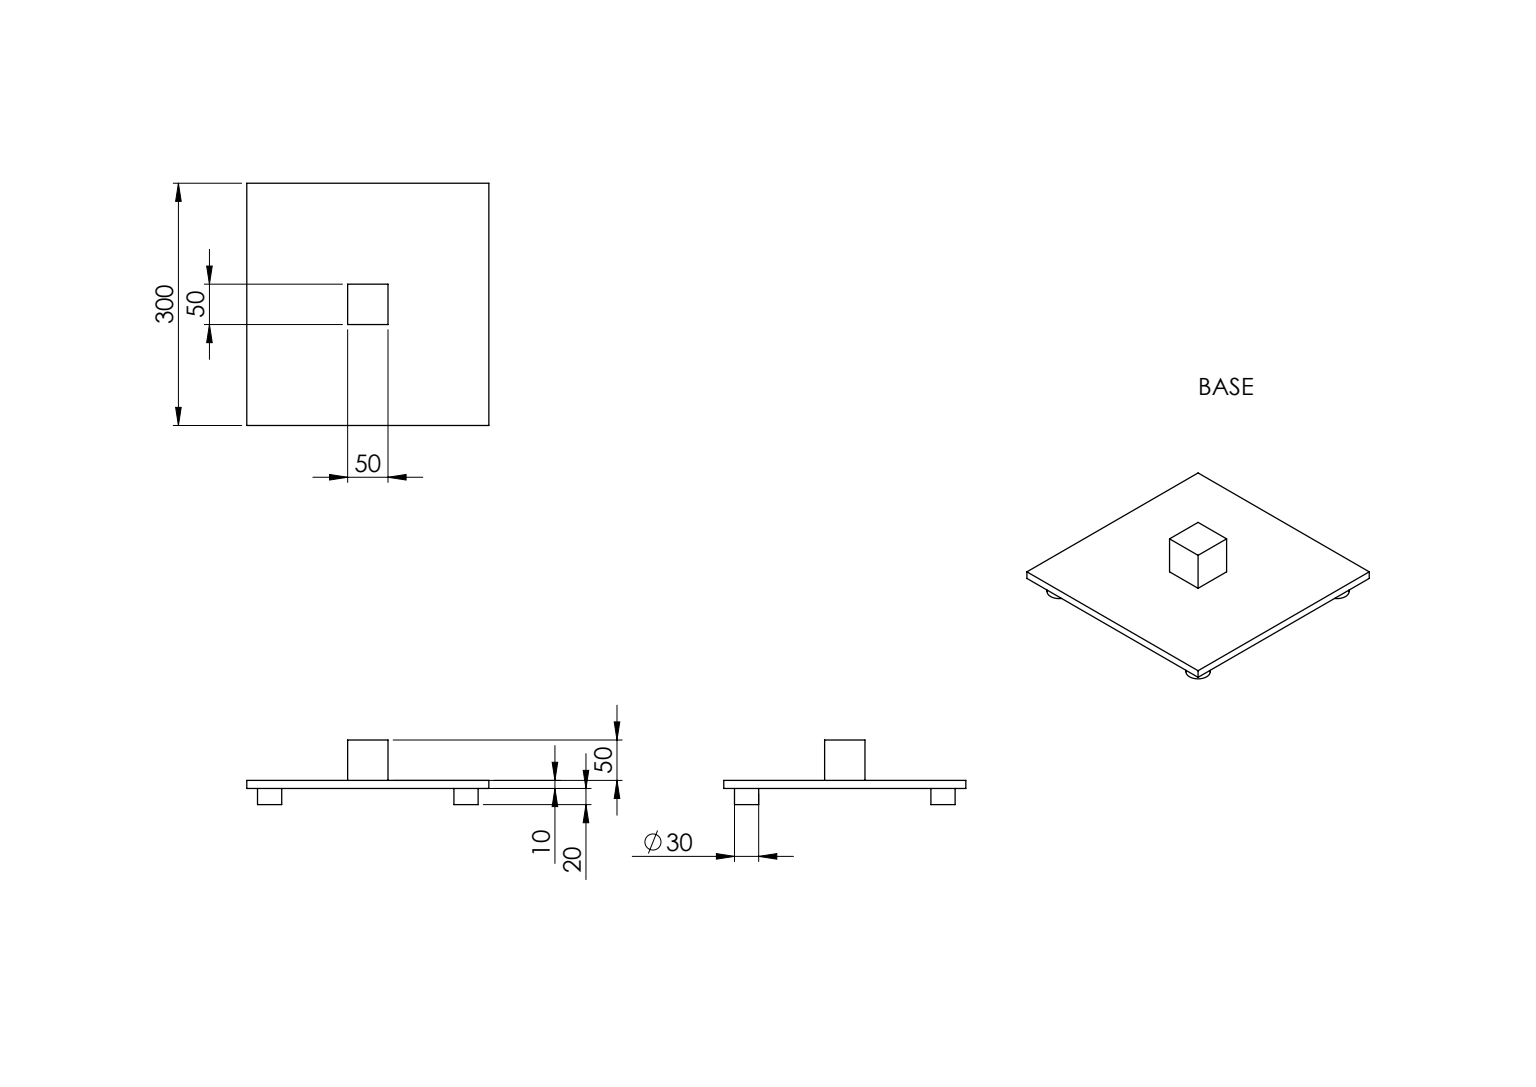
ISO-10303-21;
HEADER;
FILE_DESCRIPTION (('STEP AP214'),
    '1' );
FILE_NAME ('base.step',
    '2026-10-22T16:49:52',
    ( '' ),
    ( '' ),
    'SwSTEP 2.0',
    'SolidWorks 2026',
    '' );
FILE_SCHEMA (( 'AUTOMOTIVE_DESIGN' ));
ENDSEC;

DATA;
#2=EDGE_LOOP ( 'NONE', ( #5035, #4306, #1396, #717 ) ) ;
#9=DIRECTION ( 'NONE',  ( 1.000000000000000000, -0.000000000000000000, 0.000000000000000000 ) ) ;
#24=EDGE_LOOP ( 'NONE', ( #1798, #2180 ) ) ;
#25=CARTESIAN_POINT ( 'NONE',  ( 121.7157287525372311, 0.000000000000000000, -121.7157287525388369 ) ) ;
#29=DIRECTION ( 'NONE',  ( 0.000000000000000000, -1.000000000000000000, 0.000000000000000000 ) ) ;
#39=EDGE_CURVE ( 'NONE', #183, #4714, #3882, .T. ) ;
#40=AXIS2_PLACEMENT_3D ( 'NONE', #2568, #2148, #4717 ) ;
#42=CARTESIAN_POINT ( 'NONE',  ( 149.9999999999999716, 10.00000000000000000, 149.9999999999999716 ) ) ;
#45=EDGE_LOOP ( 'NONE', ( #4536, #2353, #4861, #2749 ) ) ;
#48=ORIENTED_EDGE ( 'NONE', *, *, #2007, .T. ) ;
#62=DIRECTION ( 'NONE',  ( -0.000000000000000000, -0.000000000000000000, 1.000000000000000000 ) ) ;
#102=CARTESIAN_POINT ( 'NONE',  ( 24.99999999999999645, 60.00000000000000711, -25.00000000000000000 ) ) ;
#108=LINE ( 'NONE', #1461, #5040 ) ;
#111=CARTESIAN_POINT ( 'NONE',  ( -150.0000000000000284, 10.00000000000000000, 149.9999999999999147 ) ) ;
#115=EDGE_CURVE ( 'NONE', #4871, #4344, #3809, .T. ) ;
#117=CARTESIAN_POINT ( 'NONE',  ( -121.7157287525381122, -20.00000000000000000, 106.7157287525380127 ) ) ;
#126=EDGE_CURVE ( 'NONE', #4344, #870, #2364, .T. ) ;
#130=AXIS2_PLACEMENT_3D ( 'NONE', #2726, #4867, #1140 ) ;
#136=EDGE_CURVE ( 'NONE', #4283, #3488, #3860, .T. ) ;
#147=CARTESIAN_POINT ( 'NONE',  ( -121.7157287525381122, 0.000000000000000000, 106.7157287525380127 ) ) ;
#154=VECTOR ( 'NONE', #5264, 1000.000000000000000 ) ;
#156=EDGE_CURVE ( 'NONE', #870, #4344, #3054, .T. ) ;
#158=LINE ( 'NONE', #4749, #4217 ) ;
#163=FACE_OUTER_BOUND ( 'NONE', #2172, .T. ) ;
#183=VERTEX_POINT ( 'NONE', #3483 ) ;
#184=CARTESIAN_POINT ( 'NONE',  ( -121.7157287525381122, 0.000000000000000000, 121.7157287525380127 ) ) ;
#188=EDGE_LOOP ( 'NONE', ( #4329, #3309, #4220, #3176 ) ) ;
#196=DIRECTION ( 'NONE',  ( -0.000000000000000000, 1.000000000000000000, -0.000000000000000000 ) ) ;
#201=CARTESIAN_POINT ( 'NONE',  ( 121.7157287525384533, -20.00000000000000000, 121.7157287525376859 ) ) ;
#212=ADVANCED_FACE ( 'NONE', ( #4821, #5247 ), #1493, .F. ) ;
#225=DIRECTION ( 'NONE',  ( -0.000000000000000000, 1.000000000000000000, -0.000000000000000000 ) ) ;
#232=VECTOR ( 'NONE', #2038, 1000.000000000000000 ) ;
#234=VECTOR ( 'NONE', #2330, 1000.000000000000000 ) ;
#254=CARTESIAN_POINT ( 'NONE',  ( -150.0000000000000284, 0.000000000000000000, 149.9999999999999147 ) ) ;
#282=LINE ( 'NONE', #1853, #2054 ) ;
#284=EDGE_CURVE ( 'NONE', #3602, #4122, #385, .T. ) ;
#285=VERTEX_POINT ( 'NONE', #3734 ) ;
#289=DIRECTION ( 'NONE',  ( 0.000000000000000000, 0.000000000000000000, 1.000000000000000000 ) ) ;
#297=DIRECTION ( 'NONE',  ( 0.000000000000000000, -1.000000000000000000, 0.000000000000000000 ) ) ;
#301=UNCERTAINTY_MEASURE_WITH_UNIT (LENGTH_MEASURE( 1.000000000000000082E-05 ), #2011, 'distance_accuracy_value', 'NONE');
#303=ORIENTED_EDGE ( 'NONE', *, *, #2481, .F. ) ;
#313=PRODUCT ( 'base', 'base', '', ( #3317 ) ) ;
#316=CARTESIAN_POINT ( 'NONE',  ( 121.7157287525384533, -20.00000000000000000, 121.7157287525376859 ) ) ;
#327=VECTOR ( 'NONE', #3004, 1000.000000000000000 ) ;
#344=FACE_OUTER_BOUND ( 'NONE', #1476, .T. ) ;
#360=ORIENTED_EDGE ( 'NONE', *, *, #1632, .T. ) ;
#377=DIRECTION ( 'NONE',  ( 0.000000000000000000, -0.000000000000000000, -1.000000000000000000 ) ) ;
#380=EDGE_CURVE ( 'NONE', #4951, #2954, #3997, .T. ) ;
#381=AXIS2_PLACEMENT_3D ( 'NONE', #2439, #1631, #3694 ) ;
#385=LINE ( 'NONE', #2047, #5346 ) ;
#392=ORIENTED_EDGE ( 'NONE', *, *, #593, .F. ) ;
#395=CIRCLE ( 'NONE', #5175, 14.99999999999998579 ) ;
#406=ORIENTED_EDGE ( 'NONE', *, *, #1500, .F. ) ;
#410=CYLINDRICAL_SURFACE ( 'NONE', #2644, 15.00000000000000000 ) ;
#420=AXIS2_PLACEMENT_3D ( 'NONE', #4558, #2003, #4859 ) ;
#430=ORIENTED_EDGE ( 'NONE', *, *, #862, .F. ) ;
#434=CARTESIAN_POINT ( 'NONE',  ( -25.00000000000000000, 60.00000000000000711, 25.00000000000000000 ) ) ;
#442=DIRECTION ( 'NONE',  ( 1.000000000000000000, 0.000000000000000000, 1.850371707708594316E-16 ) ) ;
#453=EDGE_CURVE ( 'NONE', #5233, #1447, #4280, .T. ) ;
#459=DIRECTION ( 'NONE',  ( 0.000000000000000000, -1.000000000000000000, 0.000000000000000000 ) ) ;
#462=PLANE ( 'NONE',  #2932 ) ;
#468=CIRCLE ( 'NONE', #3263, 15.00000000000000000 ) ;
#471=ADVANCED_FACE ( 'NONE', ( #519 ), #2233, .F. ) ;
#488=AXIS2_PLACEMENT_3D ( 'NONE', #3147, #2245, #5188 ) ;
#508=VERTEX_POINT ( 'NONE', #3877 ) ;
#519=FACE_OUTER_BOUND ( 'NONE', #1880, .T. ) ;
#520=CARTESIAN_POINT ( 'NONE',  ( 121.7157287525372311, -20.00000000000000000, -106.7157287525388369 ) ) ;
#523=LINE ( 'NONE', #3324, #777 ) ;
#526=CARTESIAN_POINT ( 'NONE',  ( 121.7157287525384533, -20.00000000000000000, 106.7157287525376859 ) ) ;
#529=VERTEX_POINT ( 'NONE', #4604 ) ;
#537=CARTESIAN_POINT ( 'NONE',  ( -25.00000000000000000, 10.00000000000000000, 25.00000000000000000 ) ) ;
#544=FACE_BOUND ( 'NONE', #1003, .T. ) ;
#551=CYLINDRICAL_SURFACE ( 'NONE', #3899, 15.00000000000000000 ) ;
#557=VECTOR ( 'NONE', #1931, 1000.000000000000000 ) ;
#565=PRODUCT_DEFINITION_FORMATION_WITH_SPECIFIED_SOURCE ( 'ANY', '', #313, .NOT_KNOWN. ) ;
#577=EDGE_LOOP ( 'NONE', ( #3215, #4979 ) ) ;
#589=ORIENTED_EDGE ( 'NONE', *, *, #453, .T. ) ;
#592=LINE ( 'NONE', #537, #4258 ) ;
#593=EDGE_CURVE ( 'NONE', #285, #2404, #4298, .T. ) ;
#595=ORIENTED_EDGE ( 'NONE', *, *, #3799, .F. ) ;
#596=DIRECTION ( 'NONE',  ( 0.000000000000000000, -1.000000000000000000, 0.000000000000000000 ) ) ;
#598=CARTESIAN_POINT ( 'NONE',  ( 121.7157287525384533, -20.00000000000000000, 106.7157287525376859 ) ) ;
#603=CARTESIAN_POINT ( 'NONE',  ( 25.00000000000000355, 60.00000000000000711, 25.00000000000000000 ) ) ;
#611=EDGE_CURVE ( 'NONE', #4353, #4532, #731, .T. ) ;
#623=DIRECTION ( 'NONE',  ( -1.000000000000000000, -0.000000000000000000, -0.000000000000000000 ) ) ;
#634=FACE_OUTER_BOUND ( 'NONE', #1339, .T. ) ;
#649=DIRECTION ( 'NONE',  ( 1.000000000000000000, 0.000000000000000000, -0.000000000000000000 ) ) ;
#656=VERTEX_POINT ( 'NONE', #3193 ) ;
#664=( GEOMETRIC_REPRESENTATION_CONTEXT ( 3 ) GLOBAL_UNCERTAINTY_ASSIGNED_CONTEXT ( ( #4876 ) ) GLOBAL_UNIT_ASSIGNED_CONTEXT ( ( #2048, #3372, #4579 ) ) REPRESENTATION_CONTEXT ( 'NONE', 'WORKASPACE' ) );
#665=EDGE_CURVE ( 'NONE', #5319, #2146, #4998, .T. ) ;
#685=CARTESIAN_POINT ( 'NONE',  ( 0.000000000000000000, 0.000000000000000000, 0.000000000000000000 ) ) ;
#694=DIRECTION ( 'NONE',  ( -1.000000000000000000, 0.000000000000000000, -0.000000000000000000 ) ) ;
#701=VERTEX_POINT ( 'NONE', #3518 ) ;
#703=CARTESIAN_POINT ( 'NONE',  ( -121.7157287525392917, 0.000000000000000000, -121.7157287525368332 ) ) ;
#707=( NAMED_UNIT ( * ) PLANE_ANGLE_UNIT ( ) SI_UNIT ( $, .RADIAN. ) );
#717=ORIENTED_EDGE ( 'NONE', *, *, #4118, .T. ) ;
#719=FACE_OUTER_BOUND ( 'NONE', #24, .T. ) ;
#731=CIRCLE ( 'NONE', #1938, 15.00000000000000000 ) ;
#736=CARTESIAN_POINT ( 'NONE',  ( 121.7157287525384533, 0.000000000000000000, 136.7157287525376717 ) ) ;
#738=CYLINDRICAL_SURFACE ( 'NONE', #1107, 15.00000000000000000 ) ;
#747=DIRECTION ( 'NONE',  ( 0.000000000000000000, 0.000000000000000000, 1.000000000000000000 ) ) ;
#756=CARTESIAN_POINT ( 'NONE',  ( -121.7157287525392917, -20.00000000000000000, -121.7157287525368332 ) ) ;
#769=DIRECTION ( 'NONE',  ( 1.000000000000000000, 0.000000000000000000, 0.000000000000000000 ) ) ;
#775=DIRECTION ( 'NONE',  ( 0.000000000000000000, -1.000000000000000000, 0.000000000000000000 ) ) ;
#777=VECTOR ( 'NONE', #442, 1000.000000000000000 ) ;
#799=DIRECTION ( 'NONE',  ( -1.000000000000000000, 0.000000000000000000, -9.251858538542972814E-17 ) ) ;
#804=DIRECTION ( 'NONE',  ( 0.000000000000000000, -0.000000000000000000, -1.000000000000000000 ) ) ;
#813=VERTEX_POINT ( 'NONE', #2815 ) ;
#826=AXIS2_PLACEMENT_3D ( 'NONE', #3603, #1034, #1920 ) ;
#842=EDGE_CURVE ( 'NONE', #3267, #4388, #3750, .T. ) ;
#847=AXIS2_PLACEMENT_3D ( 'NONE', #2606, #3446, #2183 ) ;
#848=ADVANCED_FACE ( 'NONE', ( #4987 ), #410, .T. ) ;
#854=DIRECTION ( 'NONE',  ( 0.000000000000000000, 0.000000000000000000, -1.000000000000000000 ) ) ;
#862=EDGE_CURVE ( 'NONE', #4388, #5233, #1567, .T. ) ;
#870=VERTEX_POINT ( 'NONE', #736 ) ;
#889=CARTESIAN_POINT ( 'NONE',  ( 0.000000000000000000, 60.00000000000000711, 0.000000000000000000 ) ) ;
#903=ORIENTED_EDGE ( 'NONE', *, *, #2485, .F. ) ;
#904=DIRECTION ( 'NONE',  ( 0.000000000000000000, 0.000000000000000000, -1.000000000000000000 ) ) ;
#908=EDGE_CURVE ( 'NONE', #4532, #4353, #4554, .T. ) ;
#917=PLANE ( 'NONE',  #130 ) ;
#925=ORIENTED_EDGE ( 'NONE', *, *, #5286, .F. ) ;
#936=VECTOR ( 'NONE', #623, 1000.000000000000000 ) ;
#938=EDGE_CURVE ( 'NONE', #3516, #2213, #468, .T. ) ;
#947=DIRECTION ( 'NONE',  ( -1.000000000000000000, 0.000000000000000000, 0.000000000000000000 ) ) ;
#955=DIRECTION ( 'NONE',  ( 0.000000000000000000, -1.000000000000000000, 0.000000000000000000 ) ) ;
#959=DIRECTION ( 'NONE',  ( -0.000000000000000000, -0.000000000000000000, 1.000000000000000000 ) ) ;
#962=VECTOR ( 'NONE', #3089, 1000.000000000000000 ) ;
#972=DIRECTION ( 'NONE',  ( -1.000000000000000000, -0.000000000000000000, -2.775557561562891351E-16 ) ) ;
#974=ORIENTED_EDGE ( 'NONE', *, *, #39, .F. ) ;
#979=PRODUCT_DEFINITION ( 'UNKNOWN', '', #565, #1182 ) ;
#997=AXIS2_PLACEMENT_3D ( 'NONE', #201, #1860, #5201 ) ;
#1003=EDGE_LOOP ( 'NONE', ( #4168, #2495 ) ) ;
#1006=CARTESIAN_POINT ( 'NONE',  ( 121.7157287525372311, -20.00000000000000000, -121.7157287525388369 ) ) ;
#1008=PLANE ( 'NONE',  #1116 ) ;
#1016=DIRECTION ( 'NONE',  ( 0.000000000000000000, 0.000000000000000000, -1.000000000000000000 ) ) ;
#1025=CARTESIAN_POINT ( 'NONE',  ( -121.7157287525381122, -20.00000000000000000, 121.7157287525380127 ) ) ;
#1029=EDGE_CURVE ( 'NONE', #2213, #3516, #1411, .T. ) ;
#1032=DIRECTION ( 'NONE',  ( -0.000000000000000000, 1.000000000000000000, -0.000000000000000000 ) ) ;
#1033=ORIENTED_EDGE ( 'NONE', *, *, #1852, .T. ) ;
#1034=DIRECTION ( 'NONE',  ( 0.000000000000000000, -1.000000000000000000, 0.000000000000000000 ) ) ;
#1035=CARTESIAN_POINT ( 'NONE',  ( -121.7157287525392917, -20.00000000000000000, -106.7157287525368332 ) ) ;
#1042=LINE ( 'NONE', #2710, #936 ) ;
#1045=EDGE_LOOP ( 'NONE', ( #5269, #1939, #430, #4843 ) ) ;
#1067=CARTESIAN_POINT ( 'NONE',  ( -121.7157287525381122, -20.00000000000000000, 106.7157287525380127 ) ) ;
#1081=EDGE_CURVE ( 'NONE', #4871, #529, #4303, .T. ) ;
#1085=ADVANCED_FACE ( 'NONE', ( #5203 ), #3984, .T. ) ;
#1088=DIRECTION ( 'NONE',  ( 0.000000000000000000, 0.000000000000000000, 1.000000000000000000 ) ) ;
#1089=FACE_OUTER_BOUND ( 'NONE', #4892, .T. ) ;
#1095=ORIENTED_EDGE ( 'NONE', *, *, #380, .F. ) ;
#1106=EDGE_CURVE ( 'NONE', #3488, #2372, #158, .T. ) ;
#1107=AXIS2_PLACEMENT_3D ( 'NONE', #3670, #2761, #1088 ) ;
#1116=AXIS2_PLACEMENT_3D ( 'NONE', #2685, #1433, #649 ) ;
#1117=ORIENTED_EDGE ( 'NONE', *, *, #39, .T. ) ;
#1132=CYLINDRICAL_SURFACE ( 'NONE', #4647, 15.00000000000000000 ) ;
#1140=DIRECTION ( 'NONE',  ( 0.000000000000000000, -0.000000000000000000, -1.000000000000000000 ) ) ;
#1166=AXIS2_PLACEMENT_3D ( 'NONE', #1842, #297, #2681 ) ;
#1168=( NAMED_UNIT ( * ) SI_UNIT ( $, .STERADIAN. ) SOLID_ANGLE_UNIT ( ) );
#1171=ORIENTED_EDGE ( 'NONE', *, *, #4109, .F. ) ;
#1182=PRODUCT_DEFINITION_CONTEXT ( 'detailed design', #4958, 'design' ) ;
#1206=LINE ( 'NONE', #2980, #232 ) ;
#1213=DIRECTION ( 'NONE',  ( 0.000000000000000000, -1.000000000000000000, 0.000000000000000000 ) ) ;
#1237=ORIENTED_EDGE ( 'NONE', *, *, #1632, .F. ) ;
#1250=DIRECTION ( 'NONE',  ( 0.000000000000000000, 0.000000000000000000, 1.000000000000000000 ) ) ;
#1273=ORIENTED_EDGE ( 'NONE', *, *, #1106, .T. ) ;
#1288=VECTOR ( 'NONE', #2476, 1000.000000000000000 ) ;
#1293=ORIENTED_EDGE ( 'NONE', *, *, #4109, .T. ) ;
#1299=CARTESIAN_POINT ( 'NONE',  ( 121.7157287525372311, -20.00000000000000000, -121.7157287525388369 ) ) ;
#1307=EDGE_LOOP ( 'NONE', ( #4818, #5283 ) ) ;
#1313=ADVANCED_FACE ( 'NONE', ( #5047 ), #462, .T. ) ;
#1319=ORIENTED_EDGE ( 'NONE', *, *, #908, .F. ) ;
#1320=CYLINDRICAL_SURFACE ( 'NONE', #3962, 15.00000000000000000 ) ;
#1334=VECTOR ( 'NONE', #3501, 1000.000000000000000 ) ;
#1338=CARTESIAN_POINT ( 'NONE',  ( 121.7157287525384533, 0.000000000000000000, 106.7157287525376859 ) ) ;
#1339=EDGE_LOOP ( 'NONE', ( #2416, #2759, #4548, #5314 ) ) ;
#1354=PRODUCT_DEFINITION_SHAPE ( 'NONE', 'NONE',  #979 ) ;
#1356=DIRECTION ( 'NONE',  ( 0.000000000000000000, -0.000000000000000000, -1.000000000000000000 ) ) ;
#1361=VECTOR ( 'NONE', #3225, 1000.000000000000000 ) ;
#1372=EDGE_LOOP ( 'NONE', ( #4478, #589, #4101, #1914 ) ) ;
#1377=EDGE_LOOP ( 'NONE', ( #2702, #5065, #3631, #3686 ) ) ;
#1380=DIRECTION ( 'NONE',  ( -2.775557561562891351E-16, 0.000000000000000000, 1.000000000000000000 ) ) ;
#1391=EDGE_LOOP ( 'NONE', ( #4455, #5173, #2058, #4539 ) ) ;
#1396=ORIENTED_EDGE ( 'NONE', *, *, #453, .F. ) ;
#1399=EDGE_CURVE ( 'NONE', #656, #2372, #5132, .T. ) ;
#1411=CIRCLE ( 'NONE', #5004, 15.00000000000000000 ) ;
#1413=LINE ( 'NONE', #2595, #4663 ) ;
#1419=CARTESIAN_POINT ( 'NONE',  ( 121.7157287525372311, -20.00000000000000000, -121.7157287525388369 ) ) ;
#1422=DIRECTION ( 'NONE',  ( -0.000000000000000000, -0.000000000000000000, 1.000000000000000000 ) ) ;
#1425=AXIS2_PLACEMENT_3D ( 'NONE', #1666, #2967, #4606 ) ;
#1432=DIRECTION ( 'NONE',  ( 0.000000000000000000, 0.000000000000000000, -1.000000000000000000 ) ) ;
#1433=DIRECTION ( 'NONE',  ( 0.000000000000000000, 0.000000000000000000, 1.000000000000000000 ) ) ;
#1445=LINE ( 'NONE', #1912, #3386 ) ;
#1447=VERTEX_POINT ( 'NONE', #4703 ) ;
#1450=ORIENTED_EDGE ( 'NONE', *, *, #4120, .F. ) ;
#1460=DIRECTION ( 'NONE',  ( 0.000000000000000000, 0.000000000000000000, -1.000000000000000000 ) ) ;
#1461=CARTESIAN_POINT ( 'NONE',  ( 149.9999999999999716, 0.000000000000000000, 149.9999999999999716 ) ) ;
#1463=LINE ( 'NONE', #3039, #2746 ) ;
#1476=EDGE_LOOP ( 'NONE', ( #3157, #4991, #5195, #4804 ) ) ;
#1479=DIRECTION ( 'NONE',  ( 1.000000000000000000, 0.000000000000000000, 1.850371707708594316E-16 ) ) ;
#1493=PLANE ( 'NONE',  #3592 ) ;
#1496=EDGE_CURVE ( 'NONE', #2213, #4532, #2628, .T. ) ;
#1499=CYLINDRICAL_SURFACE ( 'NONE', #4583, 15.00000000000000000 ) ;
#1500=EDGE_CURVE ( 'NONE', #2146, #4714, #1463, .T. ) ;
#1501=ORIENTED_EDGE ( 'NONE', *, *, #3927, .T. ) ;
#1514=FACE_BOUND ( 'NONE', #4193, .T. ) ;
#1529=MECHANICAL_DESIGN_GEOMETRIC_PRESENTATION_REPRESENTATION('',(#3380),#664);
#1530=CARTESIAN_POINT ( 'NONE',  ( -25.00000000000000000, 10.00000000000000000, 25.00000000000000000 ) ) ;
#1537=DIRECTION ( 'NONE',  ( 0.000000000000000000, -1.000000000000000000, 0.000000000000000000 ) ) ;
#1541=FILL_AREA_STYLE ('',( #4043 ) ) ;
#1559=CARTESIAN_POINT ( 'NONE',  ( -150.0000000000000284, 10.00000000000000000, 149.9999999999999147 ) ) ;
#1567=LINE ( 'NONE', #4930, #3867 ) ;
#1573=ADVANCED_FACE ( 'NONE', ( #719 ), #2415, .T. ) ;
#1582=DIRECTION ( 'NONE',  ( 0.000000000000000000, -1.000000000000000000, 0.000000000000000000 ) ) ;
#1590=( NAMED_UNIT ( * ) PLANE_ANGLE_UNIT ( ) SI_UNIT ( $, .RADIAN. ) );
#1598=CARTESIAN_POINT ( 'NONE',  ( 121.7157287525372311, 0.000000000000000000, -121.7157287525388369 ) ) ;
#1605=CARTESIAN_POINT ( 'NONE',  ( 25.00000000000000355, 10.00000000000000000, 25.00000000000000000 ) ) ;
#1609=CIRCLE ( 'NONE', #4230, 14.99999999999998579 ) ;
#1618=AXIS2_PLACEMENT_3D ( 'NONE', #4282, #2205, #1460 ) ;
#1623=ORIENTED_EDGE ( 'NONE', *, *, #3900, .F. ) ;
#1631=DIRECTION ( 'NONE',  ( 0.000000000000000000, -1.000000000000000000, 0.000000000000000000 ) ) ;
#1632=EDGE_CURVE ( 'NONE', #2355, #3602, #3201, .T. ) ;
#1646=CARTESIAN_POINT ( 'NONE',  ( 121.7157287525372311, 0.000000000000000000, -106.7157287525388369 ) ) ;
#1666=CARTESIAN_POINT ( 'NONE',  ( 0.000000000000000000, 10.00000000000000000, 0.000000000000000000 ) ) ;
#1698=CIRCLE ( 'NONE', #1948, 14.99999999999998579 ) ;
#1700=COLOUR_RGB ( '',0.8941176470588234615, 0.8941176470588234615, 0.8941176470588234615 ) ;
#1704=CLOSED_SHELL ( 'NONE', ( #4182, #4266, #848, #2419, #4143, #3046, #3376, #3139, #5154, #3778, #3323, #3865, #1313, #4477, #5357, #1813, #1573, #2678, #1085, #3540, #4827, #2531, #212, #1733, #471 ) ) ;
#1731=CARTESIAN_POINT ( 'NONE',  ( 25.00000000000000355, 60.00000000000000711, 25.00000000000000000 ) ) ;
#1733=ADVANCED_FACE ( 'NONE', ( #3490 ), #2567, .F. ) ;
#1739=CARTESIAN_POINT ( 'NONE',  ( -121.7157287525381122, -20.00000000000000000, 121.7157287525380127 ) ) ;
#1768=DIRECTION ( 'NONE',  ( 9.251858538542972814E-17, 0.000000000000000000, -1.000000000000000000 ) ) ;
#1769=AXIS2_PLACEMENT_3D ( 'NONE', #3034, #4675, #947 ) ;
#1772=DIRECTION ( 'NONE',  ( 0.000000000000000000, -1.000000000000000000, 0.000000000000000000 ) ) ;
#1774=PLANE ( 'NONE',  #4397 ) ;
#1777=VECTOR ( 'NONE', #5215, 1000.000000000000000 ) ;
#1782=( GEOMETRIC_REPRESENTATION_CONTEXT ( 3 ) GLOBAL_UNCERTAINTY_ASSIGNED_CONTEXT ( ( #301 ) ) GLOBAL_UNIT_ASSIGNED_CONTEXT ( ( #2011, #1590, #4806 ) ) REPRESENTATION_CONTEXT ( 'NONE', 'WORKASPACE' ) );
#1796=LINE ( 'NONE', #520, #3389 ) ;
#1798=ORIENTED_EDGE ( 'NONE', *, *, #2100, .T. ) ;
#1806=CARTESIAN_POINT ( 'NONE',  ( 121.7157287525384533, -20.00000000000000000, 136.7157287525376717 ) ) ;
#1813=ADVANCED_FACE ( 'NONE', ( #4863 ), #1320, .T. ) ;
#1827=EDGE_CURVE ( 'NONE', #701, #3600, #3182, .T. ) ;
#1831=LINE ( 'NONE', #3148, #234 ) ;
#1840=DIRECTION ( 'NONE',  ( -0.000000000000000000, -0.000000000000000000, 1.000000000000000000 ) ) ;
#1841=EDGE_LOOP ( 'NONE', ( #1033, #2082 ) ) ;
#1842=CARTESIAN_POINT ( 'NONE',  ( -121.7157287525392917, -20.00000000000000000, -121.7157287525368332 ) ) ;
#1848=DIRECTION ( 'NONE',  ( -1.000000000000000000, 0.000000000000000000, 1.387778780781445676E-16 ) ) ;
#1852=EDGE_CURVE ( 'NONE', #529, #4871, #2843, .T. ) ;
#1853=CARTESIAN_POINT ( 'NONE',  ( 25.00000000000000355, 60.00000000000000711, 25.00000000000000000 ) ) ;
#1860=DIRECTION ( 'NONE',  ( 0.000000000000000000, -1.000000000000000000, 0.000000000000000000 ) ) ;
#1877=ORIENTED_EDGE ( 'NONE', *, *, #842, .F. ) ;
#1880=EDGE_LOOP ( 'NONE', ( #925, #1095, #4640, #392 ) ) ;
#1887=CARTESIAN_POINT ( 'NONE',  ( -25.00000000000000000, 60.00000000000000711, 25.00000000000000000 ) ) ;
#1891=ORIENTED_EDGE ( 'NONE', *, *, #284, .F. ) ;
#1901=LINE ( 'NONE', #2406, #2958 ) ;
#1909=CYLINDRICAL_SURFACE ( 'NONE', #488, 15.00000000000000000 ) ;
#1912=CARTESIAN_POINT ( 'NONE',  ( 24.99999999999999645, 60.00000000000000711, -25.00000000000000000 ) ) ;
#1914=ORIENTED_EDGE ( 'NONE', *, *, #842, .T. ) ;
#1916=AXIS2_PLACEMENT_3D ( 'NONE', #3041, #955, #4289 ) ;
#1920=DIRECTION ( 'NONE',  ( 0.000000000000000000, -0.000000000000000000, -1.000000000000000000 ) ) ;
#1927=CARTESIAN_POINT ( 'NONE',  ( -25.00000000000000000, 60.00000000000000711, 25.00000000000000000 ) ) ;
#1931=DIRECTION ( 'NONE',  ( 1.000000000000000000, 0.000000000000000000, 0.000000000000000000 ) ) ;
#1937=EDGE_LOOP ( 'NONE', ( #4559, #1171, #5244, #1501 ) ) ;
#1938=AXIS2_PLACEMENT_3D ( 'NONE', #184, #596, #2260 ) ;
#1939=ORIENTED_EDGE ( 'NONE', *, *, #4118, .F. ) ;
#1947=EDGE_LOOP ( 'NONE', ( #2453, #4214, #4944, #595 ) ) ;
#1948=AXIS2_PLACEMENT_3D ( 'NONE', #25, #4893, #2807 ) ;
#1986=CARTESIAN_POINT ( 'NONE',  ( 121.7157287525372311, -20.00000000000000000, -121.7157287525388369 ) ) ;
#1987=DIRECTION ( 'NONE',  ( -0.000000000000000000, -1.000000000000000000, -0.000000000000000000 ) ) ;
#2003=DIRECTION ( 'NONE',  ( -0.000000000000000000, 1.000000000000000000, -0.000000000000000000 ) ) ;
#2004=ORIENTED_EDGE ( 'NONE', *, *, #3841, .F. ) ;
#2007=EDGE_CURVE ( 'NONE', #5319, #183, #3244, .T. ) ;
#2010=ORIENTED_EDGE ( 'NONE', *, *, #611, .F. ) ;
#2011=( LENGTH_UNIT ( ) NAMED_UNIT ( * ) SI_UNIT ( .MILLI., .METRE. ) );
#2030=EDGE_CURVE ( 'NONE', #2382, #813, #1698, .T. ) ;
#2037=DIRECTION ( 'NONE',  ( -0.000000000000000000, 1.000000000000000000, -0.000000000000000000 ) ) ;
#2038=DIRECTION ( 'NONE',  ( -0.000000000000000000, -1.000000000000000000, -0.000000000000000000 ) ) ;
#2039=DIRECTION ( 'NONE',  ( -9.251858538542972814E-17, 0.000000000000000000, 1.000000000000000000 ) ) ;
#2042=UNCERTAINTY_MEASURE_WITH_UNIT (LENGTH_MEASURE( 1.000000000000000082E-05 ), #4102, 'distance_accuracy_value', 'NONE');
#2044=VECTOR ( 'NONE', #4121, 1000.000000000000000 ) ;
#2046=ORIENTED_EDGE ( 'NONE', *, *, #3190, .T. ) ;
#2047=CARTESIAN_POINT ( 'NONE',  ( 25.00000000000000355, 10.00000000000000000, 25.00000000000000000 ) ) ;
#2048=( LENGTH_UNIT ( ) NAMED_UNIT ( * ) SI_UNIT ( .MILLI., .METRE. ) );
#2054=VECTOR ( 'NONE', #2249, 1000.000000000000000 ) ;
#2058=ORIENTED_EDGE ( 'NONE', *, *, #3438, .T. ) ;
#2082=ORIENTED_EDGE ( 'NONE', *, *, #1081, .T. ) ;
#2099=LINE ( 'NONE', #4994, #3097 ) ;
#2100=EDGE_CURVE ( 'NONE', #4209, #3573, #395, .T. ) ;
#2123=DIRECTION ( 'NONE',  ( -1.000000000000000000, -0.000000000000000000, -0.000000000000000000 ) ) ;
#2146=VERTEX_POINT ( 'NONE', #2537 ) ;
#2148=DIRECTION ( 'NONE',  ( 0.000000000000000000, -1.000000000000000000, 0.000000000000000000 ) ) ;
#2162=VECTOR ( 'NONE', #2123, 1000.000000000000000 ) ;
#2172=EDGE_LOOP ( 'NONE', ( #1273, #3625, #2342, #2767 ) ) ;
#2180=ORIENTED_EDGE ( 'NONE', *, *, #3245, .T. ) ;
#2183=DIRECTION ( 'NONE',  ( -1.000000000000000000, 0.000000000000000000, 0.000000000000000000 ) ) ;
#2205=DIRECTION ( 'NONE',  ( 0.000000000000000000, -1.000000000000000000, 0.000000000000000000 ) ) ;
#2213=VERTEX_POINT ( 'NONE', #117 ) ;
#2233=CYLINDRICAL_SURFACE ( 'NONE', #3417, 6.499999999999983125 ) ;
#2245=DIRECTION ( 'NONE',  ( -0.000000000000000000, 1.000000000000000000, -0.000000000000000000 ) ) ;
#2249=DIRECTION ( 'NONE',  ( -0.000000000000000000, -1.000000000000000000, -0.000000000000000000 ) ) ;
#2250=DIRECTION ( 'NONE',  ( 1.000000000000000000, 0.000000000000000000, 0.000000000000000000 ) ) ;
#2260=DIRECTION ( 'NONE',  ( 0.000000000000000000, 0.000000000000000000, -1.000000000000000000 ) ) ;
#2267=CARTESIAN_POINT ( 'NONE',  ( 149.9999999999999716, 10.00000000000000000, 149.9999999999999716 ) ) ;
#2282=LINE ( 'NONE', #4671, #3311 ) ;
#2283=EDGE_CURVE ( 'NONE', #4388, #3602, #282, .T. ) ;
#2286=ORIENTED_EDGE ( 'NONE', *, *, #1399, .T. ) ;
#2330=DIRECTION ( 'NONE',  ( -0.000000000000000000, -0.000000000000000000, 1.000000000000000000 ) ) ;
#2332=DIRECTION ( 'NONE',  ( 0.000000000000000000, 0.000000000000000000, 1.000000000000000000 ) ) ;
#2342=ORIENTED_EDGE ( 'NONE', *, *, #4716, .F. ) ;
#2350=LINE ( 'NONE', #1927, #154 ) ;
#2353=ORIENTED_EDGE ( 'NONE', *, *, #136, .F. ) ;
#2354=CARTESIAN_POINT ( 'NONE',  ( -25.00000000000000000, 10.00000000000000000, 25.00000000000000000 ) ) ;
#2355=VERTEX_POINT ( 'NONE', #1530 ) ;
#2361=FACE_OUTER_BOUND ( 'NONE', #3559, .T. ) ;
#2362=EDGE_LOOP ( 'NONE', ( #974, #2920 ) ) ;
#2364=CIRCLE ( 'NONE', #2804, 15.00000000000000000 ) ;
#2372=VERTEX_POINT ( 'NONE', #3326 ) ;
#2382=VERTEX_POINT ( 'NONE', #1646 ) ;
#2389=DIRECTION ( 'NONE',  ( 0.000000000000000000, 0.000000000000000000, 1.000000000000000000 ) ) ;
#2404=VERTEX_POINT ( 'NONE', #2425 ) ;
#2406=CARTESIAN_POINT ( 'NONE',  ( 150.0000000000000000, 10.00000000000000000, -150.0000000000000000 ) ) ;
#2415=PLANE ( 'NONE',  #5008 ) ;
#2416=ORIENTED_EDGE ( 'NONE', *, *, #4972, .F. ) ;
#2419=ADVANCED_FACE ( 'NONE', ( #344 ), #1132, .T. ) ;
#2421=CIRCLE ( 'NONE', #847, 6.499999999999983125 ) ;
#2425=CARTESIAN_POINT ( 'NONE',  ( 6.499999999999981348, 35.00000000000000000, 25.00000000000000000 ) ) ;
#2426=CYLINDRICAL_SURFACE ( 'NONE', #420, 15.00000000000000000 ) ;
#2427=EDGE_LOOP ( 'NONE', ( #3156, #4006 ) ) ;
#2429=VECTOR ( 'NONE', #959, 1000.000000000000000 ) ;
#2434=CARTESIAN_POINT ( 'NONE',  ( 0.000000000000000000, 0.000000000000000000, 0.000000000000000000 ) ) ;
#2439=CARTESIAN_POINT ( 'NONE',  ( -121.7157287525381122, 0.000000000000000000, 121.7157287525380127 ) ) ;
#2442=DIRECTION ( 'NONE',  ( 0.000000000000000000, 0.000000000000000000, 1.000000000000000000 ) ) ;
#2453=ORIENTED_EDGE ( 'NONE', *, *, #3245, .F. ) ;
#2458=APPLICATION_CONTEXT ( 'automotive_design' ) ;
#2469=DIRECTION ( 'NONE',  ( 1.000000000000000000, 0.000000000000000000, 0.000000000000000000 ) ) ;
#2476=DIRECTION ( 'NONE',  ( -0.000000000000000000, -0.000000000000000000, 1.000000000000000000 ) ) ;
#2478=VERTEX_POINT ( 'NONE', #5337 ) ;
#2481=EDGE_CURVE ( 'NONE', #2146, #5319, #1609, .T. ) ;
#2484=SHAPE_REPRESENTATION_RELATIONSHIP ( 'NONE' , 'NONE' ,  #3706, #2946 ) ;
#2485=EDGE_CURVE ( 'NONE', #656, #701, #4587, .T. ) ;
#2488=DIRECTION ( 'NONE',  ( 1.000000000000000000, 0.000000000000000000, 0.000000000000000000 ) ) ;
#2491=FACE_OUTER_BOUND ( 'NONE', #45, .T. ) ;
#2495=ORIENTED_EDGE ( 'NONE', *, *, #4972, .T. ) ;
#2498=CARTESIAN_POINT ( 'NONE',  ( -6.499999999999984901, 35.00000000000000000, -25.00000000000000000 ) ) ;
#2514=EDGE_LOOP ( 'NONE', ( #360, #2646, #1877, #1293 ) ) ;
#2519=ORIENTED_EDGE ( 'NONE', *, *, #4887, .T. ) ;
#2530=DIRECTION ( 'NONE',  ( 0.000000000000000000, 0.000000000000000000, -1.000000000000000000 ) ) ;
#2531=ADVANCED_FACE ( 'NONE', ( #2585 ), #1774, .F. ) ;
#2537=CARTESIAN_POINT ( 'NONE',  ( -121.7157287525392917, -20.00000000000000000, -136.7157287525368474 ) ) ;
#2565=ORIENTED_EDGE ( 'NONE', *, *, #3260, .F. ) ;
#2567=PLANE ( 'NONE',  #4064 ) ;
#2568=CARTESIAN_POINT ( 'NONE',  ( 121.7157287525384533, -20.00000000000000000, 121.7157287525376859 ) ) ;
#2585=FACE_OUTER_BOUND ( 'NONE', #1937, .T. ) ;
#2595=CARTESIAN_POINT ( 'NONE',  ( -150.0000000000000284, 10.00000000000000000, -150.0000000000000853 ) ) ;
#2603=CARTESIAN_POINT ( 'NONE',  ( -1.676835913137321903E-15, 35.00000000000000000, 30.00000000000000711 ) ) ;
#2606=CARTESIAN_POINT ( 'NONE',  ( -1.676835913137321903E-15, 35.00000000000000000, 25.00000000000000000 ) ) ;
#2628=LINE ( 'NONE', #1067, #1777 ) ;
#2633=FACE_OUTER_BOUND ( 'NONE', #1391, .T. ) ;
#2644=AXIS2_PLACEMENT_3D ( 'NONE', #1986, #2037, #1250 ) ;
#2646=ORIENTED_EDGE ( 'NONE', *, *, #2283, .F. ) ;
#2657=CARTESIAN_POINT ( 'NONE',  ( -150.0000000000000284, 0.000000000000000000, 149.9999999999999147 ) ) ;
#2678=ADVANCED_FACE ( 'NONE', ( #5219 ), #1909, .T. ) ;
#2681=DIRECTION ( 'NONE',  ( 0.000000000000000000, 0.000000000000000000, -1.000000000000000000 ) ) ;
#2682=DIRECTION ( 'NONE',  ( 1.850371707708594316E-16, 0.000000000000000000, -1.000000000000000000 ) ) ;
#2685=CARTESIAN_POINT ( 'NONE',  ( -25.00000000000000000, 60.00000000000000711, -25.00000000000000000 ) ) ;
#2691=FACE_OUTER_BOUND ( 'NONE', #1045, .T. ) ;
#2698=DIRECTION ( 'NONE',  ( -0.000000000000000000, -0.000000000000000000, 1.000000000000000000 ) ) ;
#2701=DIRECTION ( 'NONE',  ( -1.000000000000000000, -0.000000000000000000, -2.775557561562891351E-16 ) ) ;
#2702=ORIENTED_EDGE ( 'NONE', *, *, #1496, .F. ) ;
#2710=CARTESIAN_POINT ( 'NONE',  ( -25.00000000000000000, 10.00000000000000000, -25.00000000000000000 ) ) ;
#2726=CARTESIAN_POINT ( 'NONE',  ( 121.7157287525384533, -20.00000000000000000, 121.7157287525376859 ) ) ;
#2746=VECTOR ( 'NONE', #3144, 1000.000000000000000 ) ;
#2749=ORIENTED_EDGE ( 'NONE', *, *, #4120, .T. ) ;
#2759=ORIENTED_EDGE ( 'NONE', *, *, #5286, .T. ) ;
#2761=DIRECTION ( 'NONE',  ( -0.000000000000000000, 1.000000000000000000, -0.000000000000000000 ) ) ;
#2767=ORIENTED_EDGE ( 'NONE', *, *, #136, .T. ) ;
#2797=CARTESIAN_POINT ( 'NONE',  ( -150.0000000000000284, 10.00000000000000000, -150.0000000000000853 ) ) ;
#2804=AXIS2_PLACEMENT_3D ( 'NONE', #4734, #1772, #1016 ) ;
#2807=DIRECTION ( 'NONE',  ( 0.000000000000000000, 0.000000000000000000, -1.000000000000000000 ) ) ;
#2815=CARTESIAN_POINT ( 'NONE',  ( 121.7157287525372311, 0.000000000000000000, -136.7157287525388085 ) ) ;
#2843=CIRCLE ( 'NONE', #997, 15.00000000000000000 ) ;
#2849=MECHANICAL_DESIGN_GEOMETRIC_PRESENTATION_REPRESENTATION('',(#4730),#1782);
#2850=DIRECTION ( 'NONE',  ( 0.000000000000000000, 0.000000000000000000, -1.000000000000000000 ) ) ;
#2870=AXIS2_PLACEMENT_3D ( 'NONE', #3824, #2698, #2250 ) ;
#2884=FACE_BOUND ( 'NONE', #4150, .T. ) ;
#2914=DIRECTION ( 'NONE',  ( 0.000000000000000000, -1.000000000000000000, 0.000000000000000000 ) ) ;
#2920=ORIENTED_EDGE ( 'NONE', *, *, #3190, .F. ) ;
#2925=EDGE_LOOP ( 'NONE', ( #4124, #1450, #4407, #3749 ) ) ;
#2932=AXIS2_PLACEMENT_3D ( 'NONE', #3419, #4183, #1356 ) ;
#2941=AXIS2_PLACEMENT_3D ( 'NONE', #703, #1537, #2530 ) ;
#2946=ADVANCED_BREP_SHAPE_REPRESENTATION ( '', ( #3645, #4154 ), #3368 ) ;
#2954=VERTEX_POINT ( 'NONE', #2498 ) ;
#2958=VECTOR ( 'NONE', #1987, 1000.000000000000000 ) ;
#2960=ORIENTED_EDGE ( 'NONE', *, *, #2007, .F. ) ;
#2967=DIRECTION ( 'NONE',  ( 0.000000000000000000, -1.000000000000000000, 0.000000000000000000 ) ) ;
#2968=EDGE_CURVE ( 'NONE', #3516, #4353, #2099, .T. ) ;
#2971=DIRECTION ( 'NONE',  ( 1.000000000000000000, -0.000000000000000000, 0.000000000000000000 ) ) ;
#2975=DIRECTION ( 'NONE',  ( 0.000000000000000000, 0.000000000000000000, -1.000000000000000000 ) ) ;
#2980=CARTESIAN_POINT ( 'NONE',  ( -25.00000000000000000, 60.00000000000000711, -25.00000000000000000 ) ) ;
#2983=EDGE_CURVE ( 'NONE', #2404, #285, #2421, .T. ) ;
#2997=CARTESIAN_POINT ( 'NONE',  ( -121.7157287525381122, 0.000000000000000000, 136.7157287525380127 ) ) ;
#3004=DIRECTION ( 'NONE',  ( -0.000000000000000000, -1.000000000000000000, -0.000000000000000000 ) ) ;
#3016=DIRECTION ( 'NONE',  ( 0.000000000000000000, 0.000000000000000000, -1.000000000000000000 ) ) ;
#3026=AXIS2_PLACEMENT_3D ( 'NONE', #3904, #2682, #3496 ) ;
#3033=ORIENTED_EDGE ( 'NONE', *, *, #1827, .T. ) ;
#3034=CARTESIAN_POINT ( 'NONE',  ( -1.676835913137321903E-15, 35.00000000000000000, 25.00000000000000000 ) ) ;
#3036=CARTESIAN_POINT ( 'NONE',  ( -150.0000000000000284, 10.00000000000000000, -150.0000000000000853 ) ) ;
#3039=CARTESIAN_POINT ( 'NONE',  ( -121.7157287525392917, -20.00000000000000000, -136.7157287525368190 ) ) ;
#3041=CARTESIAN_POINT ( 'NONE',  ( 121.7157287525384533, 0.000000000000000000, 121.7157287525376859 ) ) ;
#3046=ADVANCED_FACE ( 'NONE', ( #4551, #4264 ), #5028, .F. ) ;
#3054=CIRCLE ( 'NONE', #1916, 15.00000000000000000 ) ;
#3056=ORIENTED_EDGE ( 'NONE', *, *, #156, .F. ) ;
#3058=CARTESIAN_POINT ( 'NONE',  ( -25.00000000000000000, 60.00000000000000711, -25.00000000000000000 ) ) ;
#3059=CARTESIAN_POINT ( 'NONE',  ( -150.0000000000000284, 0.000000000000000000, -150.0000000000000853 ) ) ;
#3089=DIRECTION ( 'NONE',  ( -0.000000000000000000, 1.000000000000000000, -0.000000000000000000 ) ) ;
#3095=DIRECTION ( 'NONE',  ( -0.000000000000000000, -1.000000000000000000, -0.000000000000000000 ) ) ;
#3097=VECTOR ( 'NONE', #3804, 1000.000000000000000 ) ;
#3105=AXIS2_PLACEMENT_3D ( 'NONE', #603, #1848, #3528 ) ;
#3132=ORIENTED_EDGE ( 'NONE', *, *, #1106, .F. ) ;
#3139=ADVANCED_FACE ( 'NONE', ( #3581 ), #4787, .F. ) ;
#3144=DIRECTION ( 'NONE',  ( -0.000000000000000000, 1.000000000000000000, -0.000000000000000000 ) ) ;
#3147=CARTESIAN_POINT ( 'NONE',  ( -121.7157287525392917, -20.00000000000000000, -121.7157287525368332 ) ) ;
#3148=CARTESIAN_POINT ( 'NONE',  ( 6.499999999999981348, 35.00000000000000000, 30.00000000000000711 ) ) ;
#3156=ORIENTED_EDGE ( 'NONE', *, *, #665, .T. ) ;
#3157=ORIENTED_EDGE ( 'NONE', *, *, #1081, .F. ) ;
#3168=DIRECTION ( 'NONE',  ( 0.000000000000000000, 0.000000000000000000, -1.000000000000000000 ) ) ;
#3176=ORIENTED_EDGE ( 'NONE', *, *, #2968, .F. ) ;
#3182=LINE ( 'NONE', #4778, #5012 ) ;
#3190=EDGE_CURVE ( 'NONE', #4714, #183, #5190, .T. ) ;
#3193=CARTESIAN_POINT ( 'NONE',  ( 149.9999999999999716, 10.00000000000000000, 149.9999999999999716 ) ) ;
#3200=VECTOR ( 'NONE', #5218, 1000.000000000000000 ) ;
#3201=LINE ( 'NONE', #2354, #557 ) ;
#3215=ORIENTED_EDGE ( 'NONE', *, *, #2983, .T. ) ;
#3222=SURFACE_SIDE_STYLE ('',( #3692 ) ) ;
#3223=EDGE_LOOP ( 'NONE', ( #2004, #3413, #4678, #3541 ) ) ;
#3224=DIRECTION ( 'NONE',  ( -1.387778780781445676E-16, 0.000000000000000000, -1.000000000000000000 ) ) ;
#3225=DIRECTION ( 'NONE',  ( -0.000000000000000000, 1.000000000000000000, -0.000000000000000000 ) ) ;
#3237=CARTESIAN_POINT ( 'NONE',  ( -150.0000000000000284, 10.00000000000000000, 149.9999999999999147 ) ) ;
#3244=LINE ( 'NONE', #3332, #2044 ) ;
#3245=EDGE_CURVE ( 'NONE', #3573, #4209, #3543, .T. ) ;
#3260=EDGE_CURVE ( 'NONE', #813, #2382, #4658, .T. ) ;
#3263=AXIS2_PLACEMENT_3D ( 'NONE', #1739, #29, #3846 ) ;
#3267=VERTEX_POINT ( 'NONE', #3284 ) ;
#3284=CARTESIAN_POINT ( 'NONE',  ( -25.00000000000000000, 60.00000000000000711, 25.00000000000000000 ) ) ;
#3309=ORIENTED_EDGE ( 'NONE', *, *, #1496, .T. ) ;
#3311=VECTOR ( 'NONE', #1840, 1000.000000000000000 ) ;
#3317=PRODUCT_CONTEXT ( 'NONE', #2458, 'mechanical' ) ;
#3323=ADVANCED_FACE ( 'NONE', ( #4521, #3608, #1514, #2884, #1089 ), #4495, .T. ) ;
#3324=CARTESIAN_POINT ( 'NONE',  ( -150.0000000000000284, 10.00000000000000000, 149.9999999999999147 ) ) ;
#3326=CARTESIAN_POINT ( 'NONE',  ( 149.9999999999999716, 0.000000000000000000, 149.9999999999999716 ) ) ;
#3327=CARTESIAN_POINT ( 'NONE',  ( 121.7157287525372311, -20.00000000000000000, -106.7157287525388369 ) ) ;
#3332=CARTESIAN_POINT ( 'NONE',  ( -121.7157287525392917, -20.00000000000000000, -106.7157287525368332 ) ) ;
#3368=( GEOMETRIC_REPRESENTATION_CONTEXT ( 3 ) GLOBAL_UNCERTAINTY_ASSIGNED_CONTEXT ( ( #2042 ) ) GLOBAL_UNIT_ASSIGNED_CONTEXT ( ( #4102, #707, #1168 ) ) REPRESENTATION_CONTEXT ( 'NONE', 'WORKASPACE' ) );
#3372=( NAMED_UNIT ( * ) PLANE_ANGLE_UNIT ( ) SI_UNIT ( $, .RADIAN. ) );
#3376=ADVANCED_FACE ( 'NONE', ( #4413 ), #4023, .F. ) ;
#3377=ORIENTED_EDGE ( 'NONE', *, *, #2485, .T. ) ;
#3380=STYLED_ITEM('',(#5405),#3645);
#3386=VECTOR ( 'NONE', #3596, 1000.000000000000000 ) ;
#3389=VECTOR ( 'NONE', #4337, 1000.000000000000000 ) ;
#3397=AXIS2_PLACEMENT_3D ( 'NONE', #4992, #747, #2469 ) ;
#3413=ORIENTED_EDGE ( 'NONE', *, *, #2100, .F. ) ;
#3417=AXIS2_PLACEMENT_3D ( 'NONE', #2603, #62, #4696 ) ;
#3419=CARTESIAN_POINT ( 'NONE',  ( -121.7157287525381122, -20.00000000000000000, 121.7157287525380127 ) ) ;
#3438=EDGE_CURVE ( 'NONE', #529, #870, #3561, .T. ) ;
#3446=DIRECTION ( 'NONE',  ( 0.000000000000000000, 0.000000000000000000, -1.000000000000000000 ) ) ;
#3455=DIRECTION ( 'NONE',  ( -0.000000000000000000, -1.000000000000000000, -0.000000000000000000 ) ) ;
#3457=DIRECTION ( 'NONE',  ( 9.251858538542972814E-17, 0.000000000000000000, -1.000000000000000000 ) ) ;
#3465=VECTOR ( 'NONE', #972, 1000.000000000000000 ) ;
#3474=LINE ( 'NONE', #3059, #3465 ) ;
#3483=CARTESIAN_POINT ( 'NONE',  ( -121.7157287525392917, 0.000000000000000000, -106.7157287525368332 ) ) ;
#3488=VERTEX_POINT ( 'NONE', #2657 ) ;
#3490=FACE_OUTER_BOUND ( 'NONE', #1372, .T. ) ;
#3496=DIRECTION ( 'NONE',  ( -1.000000000000000000, 0.000000000000000000, -1.850371707708594316E-16 ) ) ;
#3501=DIRECTION ( 'NONE',  ( -0.000000000000000000, -1.000000000000000000, -0.000000000000000000 ) ) ;
#3516=VERTEX_POINT ( 'NONE', #4766 ) ;
#3518=CARTESIAN_POINT ( 'NONE',  ( 150.0000000000000000, 10.00000000000000000, -150.0000000000000000 ) ) ;
#3528=DIRECTION ( 'NONE',  ( 1.387778780781445676E-16, 0.000000000000000000, 1.000000000000000000 ) ) ;
#3540=ADVANCED_FACE ( 'NONE', ( #2691 ), #4347, .F. ) ;
#3541=ORIENTED_EDGE ( 'NONE', *, *, #2030, .T. ) ;
#3543=CIRCLE ( 'NONE', #3808, 14.99999999999998579 ) ;
#3559=EDGE_LOOP ( 'NONE', ( #303, #3977, #2046, #2960 ) ) ;
#3561=LINE ( 'NONE', #1806, #3200 ) ;
#3573=VERTEX_POINT ( 'NONE', #4030 ) ;
#3577=EDGE_LOOP ( 'NONE', ( #2519, #1623, #903, #2286 ) ) ;
#3581=FACE_OUTER_BOUND ( 'NONE', #2925, .T. ) ;
#3592=AXIS2_PLACEMENT_3D ( 'NONE', #5273, #3168, #694 ) ;
#3596=DIRECTION ( 'NONE',  ( -0.000000000000000000, -1.000000000000000000, -0.000000000000000000 ) ) ;
#3600=VERTEX_POINT ( 'NONE', #2797 ) ;
#3602=VERTEX_POINT ( 'NONE', #1605 ) ;
#3603=CARTESIAN_POINT ( 'NONE',  ( -121.7157287525392917, -20.00000000000000000, -121.7157287525368332 ) ) ;
#3608=FACE_BOUND ( 'NONE', #5155, .T. ) ;
#3625=ORIENTED_EDGE ( 'NONE', *, *, #1399, .F. ) ;
#3631=ORIENTED_EDGE ( 'NONE', *, *, #2968, .T. ) ;
#3640=VERTEX_POINT ( 'NONE', #4502 ) ;
#3645=MANIFOLD_SOLID_BREP ( 'Boss-Extrude3', #1704 ) ;
#3647=AXIS2_PLACEMENT_3D ( 'NONE', #685, #775, #377 ) ;
#3662=AXIS2_PLACEMENT_3D ( 'NONE', #3753, #9, #854 ) ;
#3670=CARTESIAN_POINT ( 'NONE',  ( -121.7157287525381122, -20.00000000000000000, 121.7157287525380127 ) ) ;
#3680=VECTOR ( 'NONE', #3455, 1000.000000000000000 ) ;
#3686=ORIENTED_EDGE ( 'NONE', *, *, #611, .T. ) ;
#3692=SURFACE_STYLE_FILL_AREA ( #1541 ) ;
#3694=DIRECTION ( 'NONE',  ( 0.000000000000000000, 0.000000000000000000, -1.000000000000000000 ) ) ;
#3706=SHAPE_REPRESENTATION ( 'base', ( #4154 ), #3368 ) ;
#3734=CARTESIAN_POINT ( 'NONE',  ( -6.499999999999984901, 35.00000000000000000, 25.00000000000000000 ) ) ;
#3749=ORIENTED_EDGE ( 'NONE', *, *, #3900, .T. ) ;
#3750=LINE ( 'NONE', #434, #3789 ) ;
#3753=CARTESIAN_POINT ( 'NONE',  ( -150.0000000000000284, 10.00000000000000000, 149.9999999999999147 ) ) ;
#3778=ADVANCED_FACE ( 'NONE', ( #163 ), #3931, .F. ) ;
#3787=EDGE_LOOP ( 'NONE', ( #3377, #3033, #5010, #4835 ) ) ;
#3789=VECTOR ( 'NONE', #2488, 1000.000000000000000 ) ;
#3790=DIRECTION ( 'NONE',  ( 0.000000000000000000, -1.000000000000000000, 0.000000000000000000 ) ) ;
#3795=DIRECTION ( 'NONE',  ( 0.000000000000000000, 0.000000000000000000, -1.000000000000000000 ) ) ;
#3799=EDGE_CURVE ( 'NONE', #4209, #2382, #1796, .T. ) ;
#3804=DIRECTION ( 'NONE',  ( -0.000000000000000000, 1.000000000000000000, -0.000000000000000000 ) ) ;
#3808=AXIS2_PLACEMENT_3D ( 'NONE', #1006, #5178, #1432 ) ;
#3809=LINE ( 'NONE', #526, #962 ) ;
#3814=EDGE_CURVE ( 'NONE', #508, #2478, #3474, .T. ) ;
#3824=CARTESIAN_POINT ( 'NONE',  ( -1.676835913137321903E-15, 35.00000000000000000, 30.00000000000000711 ) ) ;
#3841=EDGE_CURVE ( 'NONE', #3573, #813, #4494, .T. ) ;
#3846=DIRECTION ( 'NONE',  ( 0.000000000000000000, 0.000000000000000000, -1.000000000000000000 ) ) ;
#3860=LINE ( 'NONE', #111, #3680 ) ;
#3865=ADVANCED_FACE ( 'NONE', ( #4022 ), #738, .T. ) ;
#3867=VECTOR ( 'NONE', #3224, 1000.000000000000000 ) ;
#3877=CARTESIAN_POINT ( 'NONE',  ( 150.0000000000000000, 0.000000000000000000, -150.0000000000000000 ) ) ;
#3882=CIRCLE ( 'NONE', #2941, 14.99999999999998579 ) ;
#3899=AXIS2_PLACEMENT_3D ( 'NONE', #5189, #225, #3916 ) ;
#3900=EDGE_CURVE ( 'NONE', #701, #508, #1901, .T. ) ;
#3904=CARTESIAN_POINT ( 'NONE',  ( -150.0000000000000284, 10.00000000000000000, 149.9999999999999147 ) ) ;
#3916=DIRECTION ( 'NONE',  ( 0.000000000000000000, 0.000000000000000000, 1.000000000000000000 ) ) ;
#3927=EDGE_CURVE ( 'NONE', #1447, #3640, #1206, .T. ) ;
#3931=PLANE ( 'NONE',  #3026 ) ;
#3962=AXIS2_PLACEMENT_3D ( 'NONE', #1419, #1032, #289 ) ;
#3967=LINE ( 'NONE', #254, #2429 ) ;
#3977=ORIENTED_EDGE ( 'NONE', *, *, #1500, .T. ) ;
#3984=PLANE ( 'NONE',  #826 ) ;
#3997=CIRCLE ( 'NONE', #3397, 6.499999999999983125 ) ;
#4006=ORIENTED_EDGE ( 'NONE', *, *, #2481, .T. ) ;
#4022=FACE_OUTER_BOUND ( 'NONE', #1377, .T. ) ;
#4023=PLANE ( 'NONE',  #4582 ) ;
#4024=CARTESIAN_POINT ( 'NONE',  ( -1.676835913137321903E-15, 35.00000000000000000, -25.00000000000000000 ) ) ;
#4030=CARTESIAN_POINT ( 'NONE',  ( 121.7157287525372311, -20.00000000000000000, -136.7157287525388085 ) ) ;
#4043=FILL_AREA_STYLE_COLOUR ( '', #1700 ) ;
#4053=ORIENTED_EDGE ( 'NONE', *, *, #4953, .F. ) ;
#4062=DIRECTION ( 'NONE',  ( -0.000000000000000000, 1.000000000000000000, -0.000000000000000000 ) ) ;
#4064=AXIS2_PLACEMENT_3D ( 'NONE', #889, #2914, #4547 ) ;
#4071=DIRECTION ( 'NONE',  ( -1.387778780781445676E-16, 0.000000000000000000, -1.000000000000000000 ) ) ;
#4101=ORIENTED_EDGE ( 'NONE', *, *, #5050, .T. ) ;
#4102=( LENGTH_UNIT ( ) NAMED_UNIT ( * ) SI_UNIT ( .MILLI., .METRE. ) );
#4109=EDGE_CURVE ( 'NONE', #3267, #2355, #5068, .T. ) ;
#4118=EDGE_CURVE ( 'NONE', #5233, #4122, #1445, .T. ) ;
#4120=EDGE_CURVE ( 'NONE', #3600, #2478, #1413, .T. ) ;
#4121=DIRECTION ( 'NONE',  ( -0.000000000000000000, 1.000000000000000000, -0.000000000000000000 ) ) ;
#4122=VERTEX_POINT ( 'NONE', #5252 ) ;
#4124=ORIENTED_EDGE ( 'NONE', *, *, #3814, .T. ) ;
#4143=ADVANCED_FACE ( 'NONE', ( #4256 ), #1499, .T. ) ;
#4150=EDGE_LOOP ( 'NONE', ( #2010, #1319 ) ) ;
#4154=AXIS2_PLACEMENT_3D ( 'NONE', #2434, #5290, #769 ) ;
#4168=ORIENTED_EDGE ( 'NONE', *, *, #380, .T. ) ;
#4182=ADVANCED_FACE ( 'NONE', ( #634 ), #4426, .F. ) ;
#4183=DIRECTION ( 'NONE',  ( 0.000000000000000000, -1.000000000000000000, 0.000000000000000000 ) ) ;
#4193=EDGE_LOOP ( 'NONE', ( #3056, #5176 ) ) ;
#4198=CARTESIAN_POINT ( 'NONE',  ( -121.7157287525381122, -20.00000000000000000, 121.7157287525380127 ) ) ;
#4209=VERTEX_POINT ( 'NONE', #3327 ) ;
#4214=ORIENTED_EDGE ( 'NONE', *, *, #3841, .T. ) ;
#4217=VECTOR ( 'NONE', #1479, 1000.000000000000000 ) ;
#4220=ORIENTED_EDGE ( 'NONE', *, *, #908, .T. ) ;
#4226=PLANE ( 'NONE',  #3662 ) ;
#4230=AXIS2_PLACEMENT_3D ( 'NONE', #756, #1582, #904 ) ;
#4237=EDGE_CURVE ( 'NONE', #3600, #4283, #5280, .T. ) ;
#4256=FACE_OUTER_BOUND ( 'NONE', #188, .T. ) ;
#4258=VECTOR ( 'NONE', #1422, 1000.000000000000000 ) ;
#4264=FACE_BOUND ( 'NONE', #5216, .T. ) ;
#4266=ADVANCED_FACE ( 'NONE', ( #2361 ), #2426, .T. ) ;
#4280=LINE ( 'NONE', #3058, #2162 ) ;
#4282=CARTESIAN_POINT ( 'NONE',  ( -121.7157287525392917, 0.000000000000000000, -121.7157287525368332 ) ) ;
#4283=VERTEX_POINT ( 'NONE', #1559 ) ;
#4289=DIRECTION ( 'NONE',  ( 0.000000000000000000, 0.000000000000000000, -1.000000000000000000 ) ) ;
#4298=CIRCLE ( 'NONE', #1769, 6.499999999999983125 ) ;
#4303=CIRCLE ( 'NONE', #40, 15.00000000000000000 ) ;
#4306=ORIENTED_EDGE ( 'NONE', *, *, #3927, .F. ) ;
#4329=ORIENTED_EDGE ( 'NONE', *, *, #1029, .F. ) ;
#4337=DIRECTION ( 'NONE',  ( -0.000000000000000000, 1.000000000000000000, -0.000000000000000000 ) ) ;
#4344=VERTEX_POINT ( 'NONE', #1338 ) ;
#4347=PLANE ( 'NONE',  #3105 ) ;
#4353=VERTEX_POINT ( 'NONE', #2997 ) ;
#4388=VERTEX_POINT ( 'NONE', #1731 ) ;
#4397=AXIS2_PLACEMENT_3D ( 'NONE', #4685, #2971, #3016 ) ;
#4407=ORIENTED_EDGE ( 'NONE', *, *, #1827, .F. ) ;
#4413=FACE_OUTER_BOUND ( 'NONE', #3577, .T. ) ;
#4426=CYLINDRICAL_SURFACE ( 'NONE', #2870, 6.499999999999983125 ) ;
#4455=ORIENTED_EDGE ( 'NONE', *, *, #115, .F. ) ;
#4458=SURFACE_STYLE_USAGE ( .BOTH. , #3222 ) ;
#4473=EDGE_CURVE ( 'NONE', #2478, #3488, #3967, .T. ) ;
#4477=ADVANCED_FACE ( 'NONE', ( #2633 ), #551, .T. ) ;
#4478=ORIENTED_EDGE ( 'NONE', *, *, #862, .T. ) ;
#4483=VECTOR ( 'NONE', #3457, 1000.000000000000000 ) ;
#4490=AXIS2_PLACEMENT_3D ( 'NONE', #1598, #5237, #2850 ) ;
#4494=LINE ( 'NONE', #4785, #1361 ) ;
#4495=PLANE ( 'NONE',  #3647 ) ;
#4502=CARTESIAN_POINT ( 'NONE',  ( -25.00000000000000000, 10.00000000000000000, -25.00000000000000000 ) ) ;
#4516=ORIENTED_EDGE ( 'NONE', *, *, #3814, .F. ) ;
#4521=FACE_BOUND ( 'NONE', #2362, .T. ) ;
#4532=VERTEX_POINT ( 'NONE', #147 ) ;
#4536=ORIENTED_EDGE ( 'NONE', *, *, #4473, .T. ) ;
#4539=ORIENTED_EDGE ( 'NONE', *, *, #156, .T. ) ;
#4547=DIRECTION ( 'NONE',  ( 0.000000000000000000, 0.000000000000000000, -1.000000000000000000 ) ) ;
#4548=ORIENTED_EDGE ( 'NONE', *, *, #2983, .F. ) ;
#4551=FACE_OUTER_BOUND ( 'NONE', #3787, .T. ) ;
#4554=CIRCLE ( 'NONE', #381, 15.00000000000000000 ) ;
#4558=CARTESIAN_POINT ( 'NONE',  ( -121.7157287525392917, -20.00000000000000000, -121.7157287525368332 ) ) ;
#4559=ORIENTED_EDGE ( 'NONE', *, *, #5238, .T. ) ;
#4564=EDGE_CURVE ( 'NONE', #4951, #2404, #1831, .T. ) ;
#4579=( NAMED_UNIT ( * ) SI_UNIT ( $, .STERADIAN. ) SOLID_ANGLE_UNIT ( ) );
#4582=AXIS2_PLACEMENT_3D ( 'NONE', #4901, #799, #2039 ) ;
#4583=AXIS2_PLACEMENT_3D ( 'NONE', #1025, #196, #2332 ) ;
#4587=LINE ( 'NONE', #42, #4483 ) ;
#4604=CARTESIAN_POINT ( 'NONE',  ( 121.7157287525384533, -20.00000000000000000, 136.7157287525376717 ) ) ;
#4606=DIRECTION ( 'NONE',  ( 0.000000000000000000, -0.000000000000000000, -1.000000000000000000 ) ) ;
#4609=ORIENTED_EDGE ( 'NONE', *, *, #5238, .F. ) ;
#4640=ORIENTED_EDGE ( 'NONE', *, *, #4564, .T. ) ;
#4647=AXIS2_PLACEMENT_3D ( 'NONE', #316, #4062, #2389 ) ;
#4658=CIRCLE ( 'NONE', #4490, 14.99999999999998579 ) ;
#4663=VECTOR ( 'NONE', #3095, 1000.000000000000000 ) ;
#4671=CARTESIAN_POINT ( 'NONE',  ( -6.499999999999984901, 35.00000000000000000, 30.00000000000000711 ) ) ;
#4675=DIRECTION ( 'NONE',  ( 0.000000000000000000, 0.000000000000000000, -1.000000000000000000 ) ) ;
#4678=ORIENTED_EDGE ( 'NONE', *, *, #3799, .T. ) ;
#4685=CARTESIAN_POINT ( 'NONE',  ( -25.00000000000000000, 60.00000000000000711, 25.00000000000000000 ) ) ;
#4696=DIRECTION ( 'NONE',  ( 1.000000000000000000, 0.000000000000000000, 0.000000000000000000 ) ) ;
#4703=CARTESIAN_POINT ( 'NONE',  ( -25.00000000000000000, 60.00000000000000711, -25.00000000000000000 ) ) ;
#4714=VERTEX_POINT ( 'NONE', #5029 ) ;
#4716=EDGE_CURVE ( 'NONE', #4283, #656, #523, .T. ) ;
#4717=DIRECTION ( 'NONE',  ( 0.000000000000000000, 0.000000000000000000, -1.000000000000000000 ) ) ;
#4730=STYLED_ITEM ( 'NONE', ( #5320 ), #2946 ) ;
#4734=CARTESIAN_POINT ( 'NONE',  ( 121.7157287525384533, 0.000000000000000000, 121.7157287525376859 ) ) ;
#4749=CARTESIAN_POINT ( 'NONE',  ( -150.0000000000000284, 0.000000000000000000, 149.9999999999999147 ) ) ;
#4752=CIRCLE ( 'NONE', #5205, 6.499999999999983125 ) ;
#4760=CARTESIAN_POINT ( 'NONE',  ( 6.499999999999981348, 35.00000000000000000, -25.00000000000000000 ) ) ;
#4766=CARTESIAN_POINT ( 'NONE',  ( -121.7157287525381122, -20.00000000000000000, 136.7157287525380127 ) ) ;
#4778=CARTESIAN_POINT ( 'NONE',  ( -150.0000000000000284, 10.00000000000000000, -150.0000000000000853 ) ) ;
#4785=CARTESIAN_POINT ( 'NONE',  ( 121.7157287525372311, -20.00000000000000000, -136.7157287525388085 ) ) ;
#4787=PLANE ( 'NONE',  #5376 ) ;
#4804=ORIENTED_EDGE ( 'NONE', *, *, #3438, .F. ) ;
#4806=( NAMED_UNIT ( * ) SI_UNIT ( $, .STERADIAN. ) SOLID_ANGLE_UNIT ( ) );
#4818=ORIENTED_EDGE ( 'NONE', *, *, #938, .T. ) ;
#4821=FACE_BOUND ( 'NONE', #577, .T. ) ;
#4827=ADVANCED_FACE ( 'NONE', ( #544, #5129 ), #1008, .F. ) ;
#4835=ORIENTED_EDGE ( 'NONE', *, *, #4716, .T. ) ;
#4843=ORIENTED_EDGE ( 'NONE', *, *, #2283, .T. ) ;
#4859=DIRECTION ( 'NONE',  ( 0.000000000000000000, 0.000000000000000000, 1.000000000000000000 ) ) ;
#4861=ORIENTED_EDGE ( 'NONE', *, *, #4237, .F. ) ;
#4863=FACE_OUTER_BOUND ( 'NONE', #3223, .T. ) ;
#4867=DIRECTION ( 'NONE',  ( 0.000000000000000000, -1.000000000000000000, 0.000000000000000000 ) ) ;
#4871=VERTEX_POINT ( 'NONE', #598 ) ;
#4876=UNCERTAINTY_MEASURE_WITH_UNIT (LENGTH_MEASURE( 1.000000000000000082E-05 ), #2048, 'distance_accuracy_value', 'NONE');
#4887=EDGE_CURVE ( 'NONE', #2372, #508, #108, .T. ) ;
#4892=EDGE_LOOP ( 'NONE', ( #5341, #3132, #4907, #4516 ) ) ;
#4893=DIRECTION ( 'NONE',  ( 0.000000000000000000, -1.000000000000000000, 0.000000000000000000 ) ) ;
#4901=CARTESIAN_POINT ( 'NONE',  ( 149.9999999999999716, 10.00000000000000000, 149.9999999999999716 ) ) ;
#4907=ORIENTED_EDGE ( 'NONE', *, *, #4473, .F. ) ;
#4930=CARTESIAN_POINT ( 'NONE',  ( 25.00000000000000355, 60.00000000000000711, 25.00000000000000000 ) ) ;
#4936=SHAPE_DEFINITION_REPRESENTATION ( #1354, #3706 ) ;
#4944=ORIENTED_EDGE ( 'NONE', *, *, #3260, .T. ) ;
#4951=VERTEX_POINT ( 'NONE', #4760 ) ;
#4953=EDGE_CURVE ( 'NONE', #4122, #3640, #1042, .T. ) ;
#4958=APPLICATION_CONTEXT ( 'automotive_design' ) ;
#4972=EDGE_CURVE ( 'NONE', #2954, #4951, #4752, .T. ) ;
#4979=ORIENTED_EDGE ( 'NONE', *, *, #593, .T. ) ;
#4987=FACE_OUTER_BOUND ( 'NONE', #1947, .T. ) ;
#4991=ORIENTED_EDGE ( 'NONE', *, *, #115, .T. ) ;
#4992=CARTESIAN_POINT ( 'NONE',  ( -1.676835913137321903E-15, 35.00000000000000000, -25.00000000000000000 ) ) ;
#4994=CARTESIAN_POINT ( 'NONE',  ( -121.7157287525381122, -20.00000000000000000, 136.7157287525380127 ) ) ;
#4998=CIRCLE ( 'NONE', #1166, 14.99999999999998579 ) ;
#5004=AXIS2_PLACEMENT_3D ( 'NONE', #4198, #459, #3795 ) ;
#5008=AXIS2_PLACEMENT_3D ( 'NONE', #5352, #1213, #804 ) ;
#5010=ORIENTED_EDGE ( 'NONE', *, *, #4237, .T. ) ;
#5012=VECTOR ( 'NONE', #2701, 1000.000000000000000 ) ;
#5028=PLANE ( 'NONE',  #1425 ) ;
#5029=CARTESIAN_POINT ( 'NONE',  ( -121.7157287525392917, 0.000000000000000000, -136.7157287525368474 ) ) ;
#5035=ORIENTED_EDGE ( 'NONE', *, *, #4953, .T. ) ;
#5040=VECTOR ( 'NONE', #1768, 1000.000000000000000 ) ;
#5047=FACE_OUTER_BOUND ( 'NONE', #1307, .T. ) ;
#5050=EDGE_CURVE ( 'NONE', #1447, #3267, #2350, .T. ) ;
#5065=ORIENTED_EDGE ( 'NONE', *, *, #938, .F. ) ;
#5068=LINE ( 'NONE', #1887, #327 ) ;
#5094=ORIENTED_EDGE ( 'NONE', *, *, #2030, .F. ) ;
#5129=FACE_OUTER_BOUND ( 'NONE', #2, .T. ) ;
#5132=LINE ( 'NONE', #2267, #1334 ) ;
#5154=ADVANCED_FACE ( 'NONE', ( #2491 ), #4226, .F. ) ;
#5155=EDGE_LOOP ( 'NONE', ( #5094, #2565 ) ) ;
#5173=ORIENTED_EDGE ( 'NONE', *, *, #1852, .F. ) ;
#5175=AXIS2_PLACEMENT_3D ( 'NONE', #1299, #3790, #2975 ) ;
#5176=ORIENTED_EDGE ( 'NONE', *, *, #126, .F. ) ;
#5178=DIRECTION ( 'NONE',  ( 0.000000000000000000, -1.000000000000000000, 0.000000000000000000 ) ) ;
#5188=DIRECTION ( 'NONE',  ( 0.000000000000000000, 0.000000000000000000, 1.000000000000000000 ) ) ;
#5189=CARTESIAN_POINT ( 'NONE',  ( 121.7157287525384533, -20.00000000000000000, 121.7157287525376859 ) ) ;
#5190=CIRCLE ( 'NONE', #1618, 14.99999999999998579 ) ;
#5194=EDGE_LOOP ( 'NONE', ( #406, #5340, #48, #1117 ) ) ;
#5195=ORIENTED_EDGE ( 'NONE', *, *, #126, .T. ) ;
#5201=DIRECTION ( 'NONE',  ( 0.000000000000000000, 0.000000000000000000, -1.000000000000000000 ) ) ;
#5203=FACE_OUTER_BOUND ( 'NONE', #2427, .T. ) ;
#5204=FACE_OUTER_BOUND ( 'NONE', #1841, .T. ) ;
#5205=AXIS2_PLACEMENT_3D ( 'NONE', #4024, #2442, #5239 ) ;
#5211=DIRECTION ( 'NONE',  ( 1.000000000000000000, 0.000000000000000000, 2.775557561562891351E-16 ) ) ;
#5215=DIRECTION ( 'NONE',  ( -0.000000000000000000, 1.000000000000000000, -0.000000000000000000 ) ) ;
#5216=EDGE_LOOP ( 'NONE', ( #1891, #1237, #4609, #4053 ) ) ;
#5218=DIRECTION ( 'NONE',  ( -0.000000000000000000, 1.000000000000000000, -0.000000000000000000 ) ) ;
#5219=FACE_OUTER_BOUND ( 'NONE', #5194, .T. ) ;
#5233=VERTEX_POINT ( 'NONE', #102 ) ;
#5237=DIRECTION ( 'NONE',  ( 0.000000000000000000, -1.000000000000000000, 0.000000000000000000 ) ) ;
#5238=EDGE_CURVE ( 'NONE', #3640, #2355, #592, .T. ) ;
#5239=DIRECTION ( 'NONE',  ( 1.000000000000000000, 0.000000000000000000, 0.000000000000000000 ) ) ;
#5244=ORIENTED_EDGE ( 'NONE', *, *, #5050, .F. ) ;
#5247=FACE_OUTER_BOUND ( 'NONE', #2514, .T. ) ;
#5252=CARTESIAN_POINT ( 'NONE',  ( 24.99999999999999645, 10.00000000000000000, -25.00000000000000000 ) ) ;
#5264=DIRECTION ( 'NONE',  ( -0.000000000000000000, -0.000000000000000000, 1.000000000000000000 ) ) ;
#5269=ORIENTED_EDGE ( 'NONE', *, *, #284, .T. ) ;
#5273=CARTESIAN_POINT ( 'NONE',  ( -25.00000000000000000, 60.00000000000000711, 25.00000000000000000 ) ) ;
#5280=LINE ( 'NONE', #3237, #1288 ) ;
#5283=ORIENTED_EDGE ( 'NONE', *, *, #1029, .T. ) ;
#5286=EDGE_CURVE ( 'NONE', #2954, #285, #2282, .T. ) ;
#5290=DIRECTION ( 'NONE',  ( 0.000000000000000000, 0.000000000000000000, 1.000000000000000000 ) ) ;
#5314=ORIENTED_EDGE ( 'NONE', *, *, #4564, .F. ) ;
#5319=VERTEX_POINT ( 'NONE', #1035 ) ;
#5320=PRESENTATION_STYLE_ASSIGNMENT (( #4458 ) ) ;
#5337=CARTESIAN_POINT ( 'NONE',  ( -150.0000000000000284, 0.000000000000000000, -150.0000000000000853 ) ) ;
#5340=ORIENTED_EDGE ( 'NONE', *, *, #665, .F. ) ;
#5341=ORIENTED_EDGE ( 'NONE', *, *, #4887, .F. ) ;
#5346=VECTOR ( 'NONE', #4071, 1000.000000000000000 ) ;
#5352=CARTESIAN_POINT ( 'NONE',  ( 121.7157287525372311, -20.00000000000000000, -121.7157287525388369 ) ) ;
#5357=ADVANCED_FACE ( 'NONE', ( #5204 ), #917, .T. ) ;
#5376=AXIS2_PLACEMENT_3D ( 'NONE', #3036, #1380, #5211 ) ;
#5399=COLOUR_RGB('Dark Blue',0.08,0.2,0.34);
#5400=FILL_AREA_STYLE_COLOUR('',#5399);
#5401=FILL_AREA_STYLE('',(#5400));
#5402=SURFACE_STYLE_FILL_AREA(#5401);
#5403=SURFACE_SIDE_STYLE('',(#5402));
#5404=SURFACE_STYLE_USAGE(.BOTH.,#5403);
#5405=PRESENTATION_STYLE_ASSIGNMENT((#5404));
ENDSEC;
END-ISO-10303-21;
